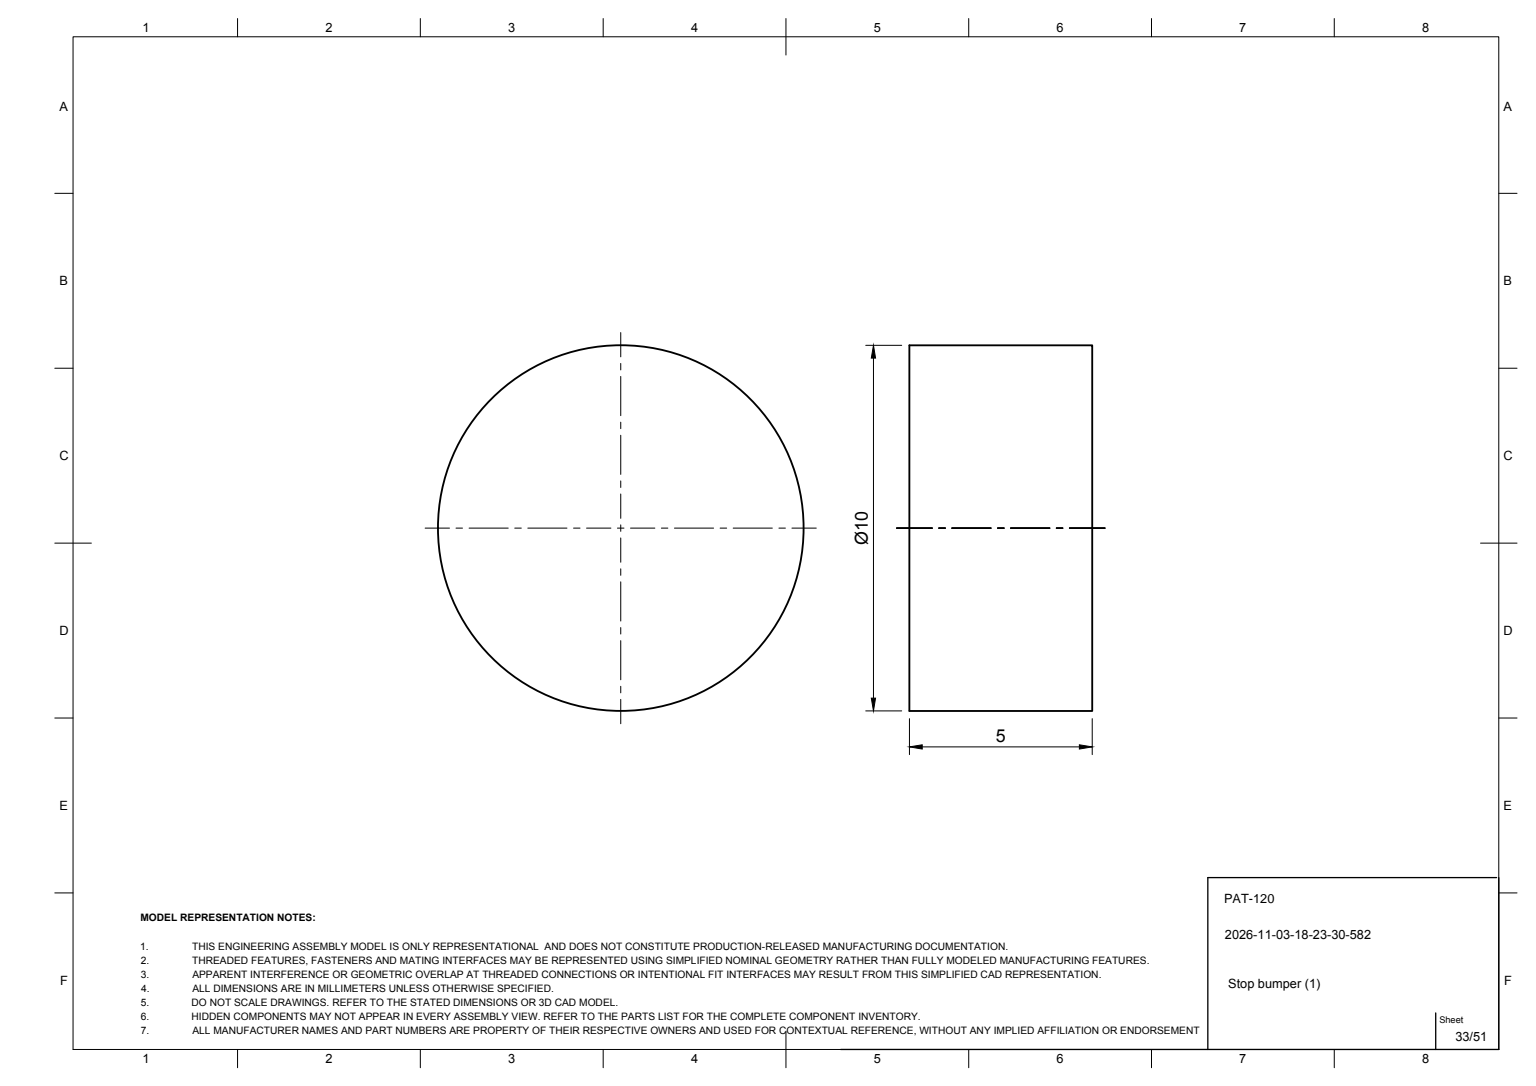
ISO-10303-21;
HEADER;
/* Generated by software containing ST-Developer
 * from STEP Tools, Inc. (www.steptools.com) 
 */

FILE_DESCRIPTION(
/* description */ ('Vibration shaker table dummy'),
/* implementation_level */ '2;1');

FILE_NAME(
/* name */ 'Stop bumper (1).step',
/* time_stamp */ '2026-10-27T10:55:14-07:00',
/* author */ (''),
/* organization */ (''),
/* preprocessor_version */ 'ST-DEVELOPER v20.2',
/* originating_system */ 'Autodesk Translation Framework v15.17.0.0',
/* authorisation */ '');

FILE_SCHEMA (('AUTOMOTIVE_DESIGN { 1 0 10303 214 3 1 1 }'));
ENDSEC;

DATA;
#10=MECHANICAL_DESIGN_GEOMETRIC_PRESENTATION_REPRESENTATION('',(#714),#22394);
#622=SHAPE_REPRESENTATION_RELATIONSHIP('SRR','None',#22668,#668);
#668=ADVANCED_BREP_SHAPE_REPRESENTATION('',(#760),#22374);
#714=STYLED_ITEM('',(#22975),#760);
#760=MANIFOLD_SOLID_BREP('Body1',#9232);
#1220=PLANE('',#10305);
#1221=PLANE('',#10306);
#1614=FACE_OUTER_BOUND('',#2282,.T.);
#1615=FACE_OUTER_BOUND('',#2283,.T.);
#1616=FACE_OUTER_BOUND('',#2284,.T.);
#2282=EDGE_LOOP('',(#7452,#7453,#7454,#7455));
#2283=EDGE_LOOP('',(#7456));
#2284=EDGE_LOOP('',(#7457));
#2979=LINE('',#21040,#3598);
#3598=VECTOR('',#12395,0.5);
#4102=CIRCLE('',#10303,0.5);
#4103=CIRCLE('',#10304,0.5);
#4769=VERTEX_POINT('',#21037);
#4770=VERTEX_POINT('',#21039);
#5719=EDGE_CURVE('',#4769,#4769,#4102,.T.);
#5720=EDGE_CURVE('',#4769,#4770,#2979,.T.);
#5721=EDGE_CURVE('',#4770,#4770,#4103,.T.);
#7452=ORIENTED_EDGE('',*,*,#5719,.F.);
#7453=ORIENTED_EDGE('',*,*,#5720,.T.);
#7454=ORIENTED_EDGE('',*,*,#5721,.T.);
#7455=ORIENTED_EDGE('',*,*,#5720,.F.);
#7456=ORIENTED_EDGE('',*,*,#5719,.T.);
#7457=ORIENTED_EDGE('',*,*,#5721,.F.);
#8615=CYLINDRICAL_SURFACE('',#10302,0.5);
#8979=ADVANCED_FACE('',(#1614),#8615,.T.);
#8980=ADVANCED_FACE('',(#1615),#1220,.T.);
#8981=ADVANCED_FACE('',(#1616),#1221,.F.);
#9232=CLOSED_SHELL('',(#8979,#8980,#8981));
#10301=AXIS2_PLACEMENT_3D('',#21035,#12389,#12390);
#10302=AXIS2_PLACEMENT_3D('',#21036,#12391,#12392);
#10303=AXIS2_PLACEMENT_3D('',#21038,#12393,#12394);
#10304=AXIS2_PLACEMENT_3D('',#21041,#12396,#12397);
#10305=AXIS2_PLACEMENT_3D('',#21042,#12398,#12399);
#10306=AXIS2_PLACEMENT_3D('',#21043,#12400,#12401);
#12389=DIRECTION('axis',(0.,0.,1.));
#12390=DIRECTION('refdir',(1.,0.,0.));
#12391=DIRECTION('center_axis',(0.,0.,1.));
#12392=DIRECTION('ref_axis',(1.,0.,0.));
#12393=DIRECTION('center_axis',(0.,0.,1.));
#12394=DIRECTION('ref_axis',(1.,0.,0.));
#12395=DIRECTION('',(0.,0.,-1.));
#12396=DIRECTION('center_axis',(0.,0.,1.));
#12397=DIRECTION('ref_axis',(1.,0.,0.));
#12398=DIRECTION('center_axis',(0.,0.,1.));
#12399=DIRECTION('ref_axis',(1.,0.,0.));
#12400=DIRECTION('center_axis',(0.,0.,1.));
#12401=DIRECTION('ref_axis',(1.,0.,0.));
#21035=CARTESIAN_POINT('',(0.,0.,0.));
#21036=CARTESIAN_POINT('Origin',(0.,-6.,17.3));
#21037=CARTESIAN_POINT('',(-0.5,-6.,17.8));
#21038=CARTESIAN_POINT('Origin',(0.,-6.,17.8));
#21039=CARTESIAN_POINT('',(-0.5,-6.,17.3));
#21040=CARTESIAN_POINT('',(-0.5,-6.,17.3));
#21041=CARTESIAN_POINT('Origin',(0.,-6.,17.3));
#21042=CARTESIAN_POINT('Origin',(0.,-6.,17.8));
#21043=CARTESIAN_POINT('Origin',(0.,-6.,17.3));
#22323=UNCERTAINTY_MEASURE_WITH_UNIT(LENGTH_MEASURE(0.001),#22395,
'DISTANCE_ACCURACY_VALUE',
'Maximum model space distance between geometric entities at asserted c
onnectivities');
#22343=UNCERTAINTY_MEASURE_WITH_UNIT(LENGTH_MEASURE(0.001),#22395,
'DISTANCE_ACCURACY_VALUE',
'Maximum model space distance between geometric entities at asserted c
onnectivities');
#22374=(
GEOMETRIC_REPRESENTATION_CONTEXT(3)
GLOBAL_UNCERTAINTY_ASSIGNED_CONTEXT((#22323))
GLOBAL_UNIT_ASSIGNED_CONTEXT((#22395,#22397,#22398))
REPRESENTATION_CONTEXT('','3D')
);
#22394=(
GEOMETRIC_REPRESENTATION_CONTEXT(3)
GLOBAL_UNCERTAINTY_ASSIGNED_CONTEXT((#22343))
GLOBAL_UNIT_ASSIGNED_CONTEXT((#22395,#22397,#22398))
REPRESENTATION_CONTEXT('','3D')
);
#22395=(
LENGTH_UNIT()
NAMED_UNIT(*)
SI_UNIT(.CENTI.,.METRE.)
);
#22397=(
NAMED_UNIT(*)
PLANE_ANGLE_UNIT()
SI_UNIT($,.RADIAN.)
);
#22398=(
NAMED_UNIT(*)
SI_UNIT($,.STERADIAN.)
SOLID_ANGLE_UNIT()
);
#22429=SHAPE_DEFINITION_REPRESENTATION(#22479,#22668);
#22479=PRODUCT_DEFINITION_SHAPE('',$,#22719);
#22668=SHAPE_REPRESENTATION('',(#10301),#22374);
#22688=PRODUCT_DEFINITION_CONTEXT('part definition',#22840,'design');
#22719=PRODUCT_DEFINITION('Stop bumper (1)','Stop bumper (1)',#22769,#22688);
#22769=PRODUCT_DEFINITION_FORMATION('',$,#22872);
#22840=APPLICATION_CONTEXT(
'Core Data for Automotive Mechanical Design Process');
#22841=PRODUCT_CONTEXT('part definition',#22840,'mechanical');
#22872=PRODUCT('Stop bumper (1)','Stop bumper (1)','Stop bumper (1)',(#22841));
#22969=COLOUR_RGB('Off White',0.89,0.88,0.83);
#22970=FILL_AREA_STYLE_COLOUR('',#22969);
#22971=FILL_AREA_STYLE('',(#22970));
#22972=SURFACE_STYLE_FILL_AREA(#22971);
#22973=SURFACE_SIDE_STYLE('',(#22972));
#22974=SURFACE_STYLE_USAGE(.BOTH.,#22973);
#22975=PRESENTATION_STYLE_ASSIGNMENT((#22974));
ENDSEC;
END-ISO-10303-21;
